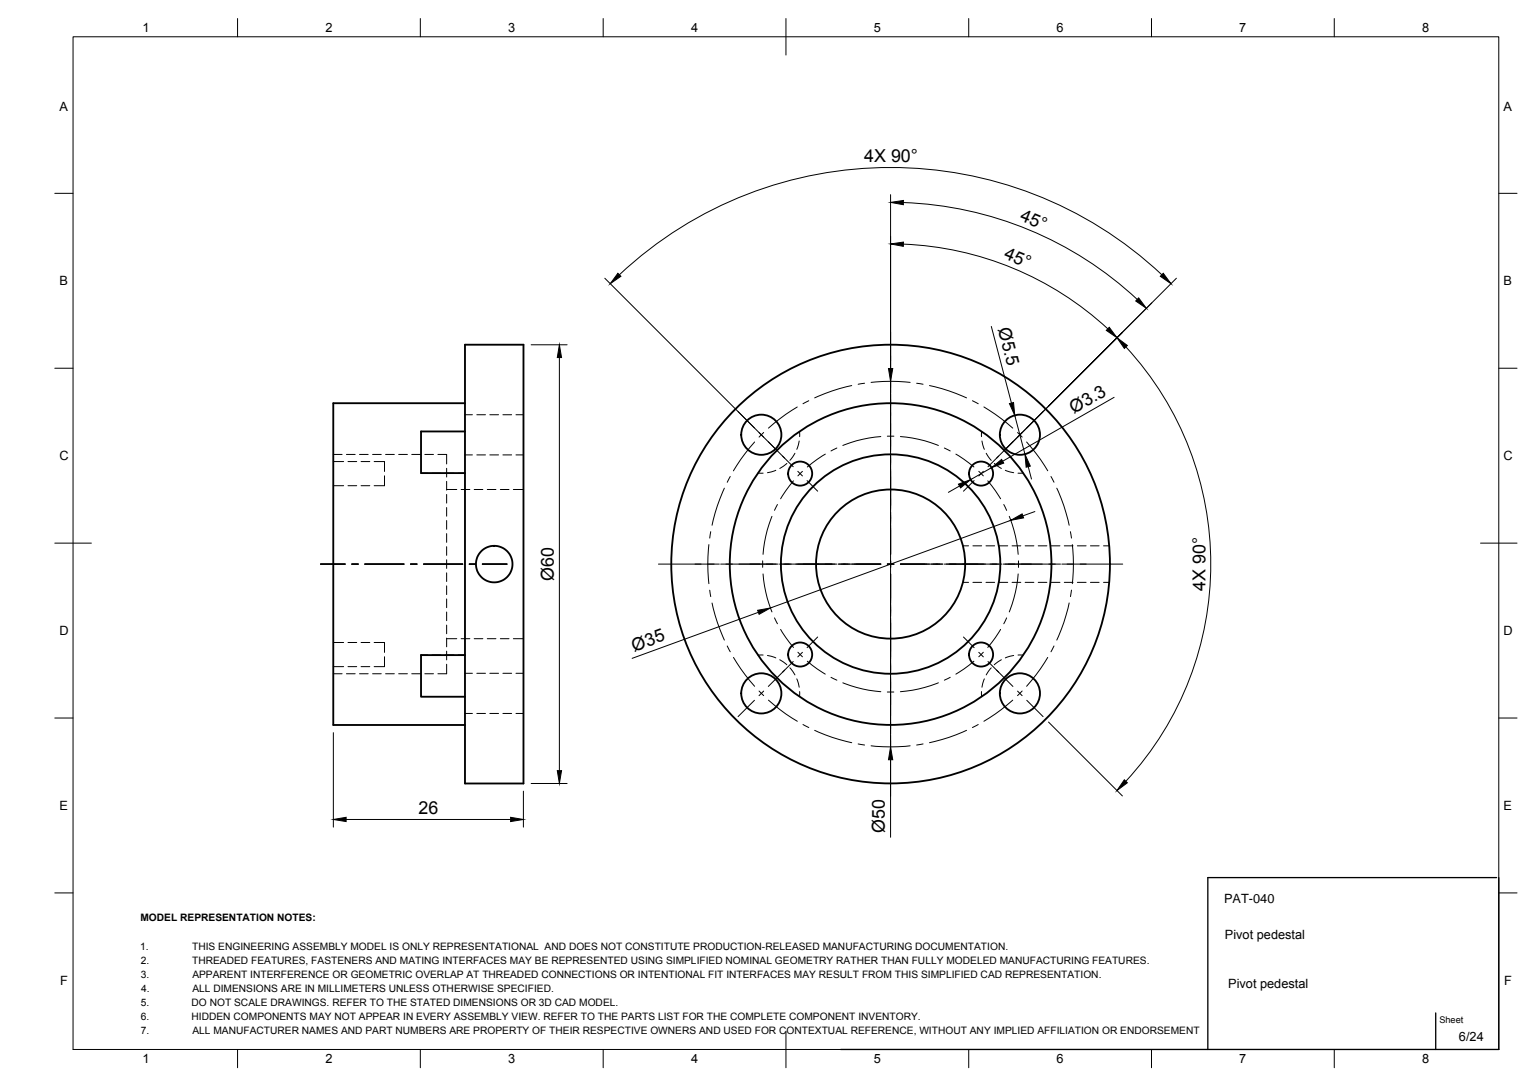
ISO-10303-21;
HEADER;
/* Generated by software containing ST-Developer
 * from STEP Tools, Inc. (www.steptools.com) 
 */

FILE_DESCRIPTION(
/* description */ ('Four-bar tabletop demonstrator'),
/* implementation_level */ '2;1');

FILE_NAME(
/* name */ 'Pivot pedestal.step',
/* time_stamp */ '2026-10-29T17:05:23-07:00',
/* author */ (''),
/* organization */ (''),
/* preprocessor_version */ 'ST-DEVELOPER v20.2',
/* originating_system */ 'Autodesk Translation Framework v15.17.0.0',
/* authorisation */ '');

FILE_SCHEMA (('AUTOMOTIVE_DESIGN { 1 0 10303 214 3 1 1 }'));
ENDSEC;

DATA;
#10=MECHANICAL_DESIGN_GEOMETRIC_PRESENTATION_REPRESENTATION('',(#338),#6705);
#280=B_SPLINE_CURVE_WITH_KNOTS('',3,(#5305,#5306,#5307,#5308,#5309,#5310,
#5311,#5312,#5313,#5314),.UNSPECIFIED.,.F.,.F.,(4,2,2,2,4),(0.,0.0945941824764479,
0.189188364952896,0.283770357603024,0.378352350253152),.UNSPECIFIED.);
#281=B_SPLINE_CURVE_WITH_KNOTS('',3,(#5315,#5316,#5317,#5318,#5319,#5320,
#5321,#5322,#5323,#5324,#5325,#5326,#5327,#5328,#5329,#5330,#5331,#5332,
#5333,#5334,#5335,#5336,#5337,#5338,#5339,#5340),.UNSPECIFIED.,.F.,.F.,
(4,2,2,2,2,2,2,2,2,2,2,2,4),(0.378352350253152,0.47293434290328,0.567516335553408,
0.662110518029855,0.756704700506303,0.851298882982751,0.945893065459199,
1.04047505810933,1.13505705075946,1.22963904340958,1.32422103605971,1.41881521853616,
1.51340940101261),.UNSPECIFIED.);
#282=B_SPLINE_CURVE_WITH_KNOTS('',3,(#5344,#5345,#5346,#5347,#5348,#5349,
#5350,#5351,#5352,#5353,#5354,#5355,#5356,#5357,#5358,#5359,#5360,#5361,
#5362,#5363,#5364,#5365,#5366,#5367,#5368,#5369),.UNSPECIFIED.,.F.,.F.,
(4,2,2,2,2,2,2,2,2,2,2,2,4),(0.,0.0942186410044058,0.188437282008812,0.282655768798837,
0.376874255588861,0.471092742378886,0.565311229168911,0.659529870173317,
0.753748511177723,0.847967152182129,0.942185793186535,1.03640427997656,
1.13062276676658),.UNSPECIFIED.);
#283=B_SPLINE_CURVE_WITH_KNOTS('',3,(#5370,#5371,#5372,#5373,#5374,#5375,
#5376,#5377,#5378,#5379),.UNSPECIFIED.,.F.,.F.,(4,2,2,2,4),(1.13062276676658,
1.22484125355661,1.31905974034663,1.41327838135104,1.50749702235545),
 .UNSPECIFIED.);
#308=SHAPE_REPRESENTATION_RELATIONSHIP('SRR','None',#6814,#323);
#323=ADVANCED_BREP_SHAPE_REPRESENTATION('',(#361),#6687);
#338=STYLED_ITEM('',(#7003),#361);
#361=MANIFOLD_SOLID_BREP('Body1',#3382);
#397=FACE_BOUND('',#814,.T.);
#398=FACE_BOUND('',#815,.T.);
#399=FACE_BOUND('',#816,.T.);
#400=FACE_BOUND('',#817,.T.);
#401=FACE_BOUND('',#818,.T.);
#402=FACE_BOUND('',#825,.T.);
#403=FACE_BOUND('',#827,.T.);
#404=FACE_BOUND('',#829,.T.);
#405=FACE_BOUND('',#831,.T.);
#406=FACE_BOUND('',#832,.T.);
#407=FACE_BOUND('',#833,.T.);
#408=FACE_BOUND('',#834,.T.);
#409=FACE_BOUND('',#835,.T.);
#410=FACE_BOUND('',#837,.T.);
#411=FACE_BOUND('',#838,.T.);
#412=FACE_BOUND('',#839,.T.);
#413=FACE_BOUND('',#840,.T.);
#414=FACE_BOUND('',#841,.T.);
#468=PLANE('',#3610);
#469=PLANE('',#3614);
#470=PLANE('',#3618);
#471=PLANE('',#3622);
#472=PLANE('',#3623);
#473=PLANE('',#3631);
#474=PLANE('',#3636);
#475=PLANE('',#3641);
#476=PLANE('',#3650);
#477=PLANE('',#3667);
#478=PLANE('',#3673);
#479=PLANE('',#3674);
#576=FACE_OUTER_BOUND('',#795,.T.);
#577=FACE_OUTER_BOUND('',#796,.T.);
#578=FACE_OUTER_BOUND('',#797,.T.);
#579=FACE_OUTER_BOUND('',#798,.T.);
#580=FACE_OUTER_BOUND('',#799,.T.);
#581=FACE_OUTER_BOUND('',#800,.T.);
#582=FACE_OUTER_BOUND('',#801,.T.);
#583=FACE_OUTER_BOUND('',#802,.T.);
#584=FACE_OUTER_BOUND('',#803,.T.);
#585=FACE_OUTER_BOUND('',#804,.T.);
#586=FACE_OUTER_BOUND('',#805,.T.);
#587=FACE_OUTER_BOUND('',#806,.T.);
#588=FACE_OUTER_BOUND('',#807,.T.);
#589=FACE_OUTER_BOUND('',#808,.T.);
#590=FACE_OUTER_BOUND('',#809,.T.);
#591=FACE_OUTER_BOUND('',#810,.T.);
#592=FACE_OUTER_BOUND('',#811,.T.);
#593=FACE_OUTER_BOUND('',#812,.T.);
#594=FACE_OUTER_BOUND('',#813,.T.);
#595=FACE_OUTER_BOUND('',#819,.T.);
#596=FACE_OUTER_BOUND('',#820,.T.);
#597=FACE_OUTER_BOUND('',#821,.T.);
#598=FACE_OUTER_BOUND('',#822,.T.);
#599=FACE_OUTER_BOUND('',#823,.T.);
#600=FACE_OUTER_BOUND('',#824,.T.);
#601=FACE_OUTER_BOUND('',#826,.T.);
#602=FACE_OUTER_BOUND('',#828,.T.);
#603=FACE_OUTER_BOUND('',#830,.T.);
#604=FACE_OUTER_BOUND('',#836,.T.);
#795=EDGE_LOOP('',(#2360,#2361,#2362,#2363,#2364,#2365));
#796=EDGE_LOOP('',(#2366,#2367,#2368,#2369));
#797=EDGE_LOOP('',(#2370));
#798=EDGE_LOOP('',(#2371,#2372,#2373,#2374));
#799=EDGE_LOOP('',(#2375));
#800=EDGE_LOOP('',(#2376,#2377,#2378,#2379));
#801=EDGE_LOOP('',(#2380));
#802=EDGE_LOOP('',(#2381,#2382,#2383,#2384));
#803=EDGE_LOOP('',(#2385));
#804=EDGE_LOOP('',(#2386,#2387));
#805=EDGE_LOOP('',(#2388,#2389,#2390,#2391));
#806=EDGE_LOOP('',(#2392,#2393,#2394,#2395));
#807=EDGE_LOOP('',(#2396,#2397));
#808=EDGE_LOOP('',(#2398,#2399,#2400,#2401));
#809=EDGE_LOOP('',(#2402,#2403));
#810=EDGE_LOOP('',(#2404,#2405,#2406,#2407));
#811=EDGE_LOOP('',(#2408,#2409));
#812=EDGE_LOOP('',(#2410,#2411,#2412,#2413,#2414,#2415,#2416,#2417,#2418,
#2419,#2420,#2421,#2422,#2423,#2424,#2425,#2426,#2427,#2428,#2429));
#813=EDGE_LOOP('',(#2430));
#814=EDGE_LOOP('',(#2431,#2432,#2433,#2434,#2435,#2436,#2437,#2438,#2439));
#815=EDGE_LOOP('',(#2440));
#816=EDGE_LOOP('',(#2441));
#817=EDGE_LOOP('',(#2442));
#818=EDGE_LOOP('',(#2443));
#819=EDGE_LOOP('',(#2444,#2445,#2446,#2447));
#820=EDGE_LOOP('',(#2448,#2449,#2450,#2451));
#821=EDGE_LOOP('',(#2452,#2453,#2454,#2455));
#822=EDGE_LOOP('',(#2456,#2457,#2458,#2459));
#823=EDGE_LOOP('',(#2460,#2461,#2462,#2463));
#824=EDGE_LOOP('',(#2464));
#825=EDGE_LOOP('',(#2465));
#826=EDGE_LOOP('',(#2466,#2467,#2468,#2469));
#827=EDGE_LOOP('',(#2470,#2471));
#828=EDGE_LOOP('',(#2472,#2473,#2474,#2475));
#829=EDGE_LOOP('',(#2476,#2477));
#830=EDGE_LOOP('',(#2478));
#831=EDGE_LOOP('',(#2479));
#832=EDGE_LOOP('',(#2480));
#833=EDGE_LOOP('',(#2481));
#834=EDGE_LOOP('',(#2482));
#835=EDGE_LOOP('',(#2483));
#836=EDGE_LOOP('',(#2484));
#837=EDGE_LOOP('',(#2485));
#838=EDGE_LOOP('',(#2486));
#839=EDGE_LOOP('',(#2487));
#840=EDGE_LOOP('',(#2488));
#841=EDGE_LOOP('',(#2489));
#1069=LINE('',#5342,#1239);
#1070=LINE('',#5384,#1240);
#1071=LINE('',#5391,#1241);
#1072=LINE('',#5398,#1242);
#1073=LINE('',#5405,#1243);
#1074=LINE('',#5415,#1244);
#1075=LINE('',#5418,#1245);
#1076=LINE('',#5422,#1246);
#1077=LINE('',#5426,#1247);
#1078=LINE('',#5433,#1248);
#1079=LINE('',#5437,#1249);
#1080=LINE('',#5444,#1250);
#1081=LINE('',#5448,#1251);
#1082=LINE('',#5456,#1252);
#1083=LINE('',#5476,#1253);
#1084=LINE('',#5480,#1254);
#1085=LINE('',#5484,#1255);
#1086=LINE('',#5488,#1256);
#1087=LINE('',#5493,#1257);
#1088=LINE('',#5500,#1258);
#1089=LINE('',#5504,#1259);
#1239=VECTOR('',#4156,0.25);
#1240=VECTOR('',#4161,0.165);
#1241=VECTOR('',#4170,0.165);
#1242=VECTOR('',#4179,0.165);
#1243=VECTOR('',#4188,0.165);
#1244=VECTOR('',#4201,1.);
#1245=VECTOR('',#4204,1.);
#1246=VECTOR('',#4207,1.);
#1247=VECTOR('',#4210,1.);
#1248=VECTOR('',#4219,1.);
#1249=VECTOR('',#4222,1.);
#1250=VECTOR('',#4231,1.);
#1251=VECTOR('',#4234,1.);
#1252=VECTOR('',#4245,2.2);
#1253=VECTOR('',#4272,0.275);
#1254=VECTOR('',#4277,0.275);
#1255=VECTOR('',#4282,0.275);
#1256=VECTOR('',#4287,0.275);
#1257=VECTOR('',#4292,1.5);
#1258=VECTOR('',#4301,3.);
#1259=VECTOR('',#4306,1.02);
#1405=CIRCLE('',#3608,0.165);
#1406=CIRCLE('',#3609,0.165);
#1407=CIRCLE('',#3612,0.165);
#1408=CIRCLE('',#3613,0.165);
#1409=CIRCLE('',#3616,0.165);
#1410=CIRCLE('',#3617,0.165);
#1411=CIRCLE('',#3620,0.165);
#1412=CIRCLE('',#3621,0.165);
#1413=CIRCLE('',#3624,2.2);
#1414=CIRCLE('',#3625,0.525);
#1415=CIRCLE('',#3627,0.525);
#1416=CIRCLE('',#3629,0.525);
#1417=CIRCLE('',#3630,0.525);
#1418=CIRCLE('',#3632,2.2);
#1419=CIRCLE('',#3634,0.525);
#1420=CIRCLE('',#3635,0.525);
#1421=CIRCLE('',#3637,2.2);
#1422=CIRCLE('',#3639,0.525);
#1423=CIRCLE('',#3640,0.525);
#1424=CIRCLE('',#3642,2.2);
#1425=CIRCLE('',#3644,2.2);
#1426=CIRCLE('',#3645,2.2);
#1427=CIRCLE('',#3646,2.2);
#1428=CIRCLE('',#3647,2.2);
#1429=CIRCLE('',#3648,2.2);
#1430=CIRCLE('',#3649,2.2);
#1431=CIRCLE('',#3651,3.);
#1432=CIRCLE('',#3652,0.275);
#1433=CIRCLE('',#3653,0.275);
#1434=CIRCLE('',#3654,0.275);
#1435=CIRCLE('',#3655,0.275);
#1436=CIRCLE('',#3657,0.275);
#1437=CIRCLE('',#3659,0.275);
#1438=CIRCLE('',#3661,0.275);
#1439=CIRCLE('',#3663,0.275);
#1440=CIRCLE('',#3665,1.5);
#1441=CIRCLE('',#3666,1.5);
#1442=CIRCLE('',#3668,1.02);
#1443=CIRCLE('',#3670,3.);
#1444=CIRCLE('',#3672,1.02);
#1624=VERTEX_POINT('',#5303);
#1625=VERTEX_POINT('',#5304);
#1626=VERTEX_POINT('',#5341);
#1627=VERTEX_POINT('',#5343);
#1628=VERTEX_POINT('',#5381);
#1629=VERTEX_POINT('',#5383);
#1630=VERTEX_POINT('',#5388);
#1631=VERTEX_POINT('',#5390);
#1632=VERTEX_POINT('',#5395);
#1633=VERTEX_POINT('',#5397);
#1634=VERTEX_POINT('',#5402);
#1635=VERTEX_POINT('',#5404);
#1636=VERTEX_POINT('',#5409);
#1637=VERTEX_POINT('',#5410);
#1638=VERTEX_POINT('',#5414);
#1639=VERTEX_POINT('',#5416);
#1640=VERTEX_POINT('',#5420);
#1641=VERTEX_POINT('',#5421);
#1642=VERTEX_POINT('',#5423);
#1643=VERTEX_POINT('',#5425);
#1644=VERTEX_POINT('',#5431);
#1645=VERTEX_POINT('',#5432);
#1646=VERTEX_POINT('',#5434);
#1647=VERTEX_POINT('',#5436);
#1648=VERTEX_POINT('',#5442);
#1649=VERTEX_POINT('',#5443);
#1650=VERTEX_POINT('',#5445);
#1651=VERTEX_POINT('',#5447);
#1652=VERTEX_POINT('',#5453);
#1653=VERTEX_POINT('',#5455);
#1654=VERTEX_POINT('',#5463);
#1655=VERTEX_POINT('',#5465);
#1656=VERTEX_POINT('',#5467);
#1657=VERTEX_POINT('',#5469);
#1658=VERTEX_POINT('',#5471);
#1659=VERTEX_POINT('',#5474);
#1660=VERTEX_POINT('',#5478);
#1661=VERTEX_POINT('',#5482);
#1662=VERTEX_POINT('',#5486);
#1663=VERTEX_POINT('',#5490);
#1664=VERTEX_POINT('',#5492);
#1665=VERTEX_POINT('',#5496);
#1666=VERTEX_POINT('',#5499);
#1667=VERTEX_POINT('',#5503);
#1916=EDGE_CURVE('',#1624,#1625,#280,.T.);
#1917=EDGE_CURVE('',#1625,#1624,#281,.T.);
#1918=EDGE_CURVE('',#1625,#1626,#1069,.T.);
#1919=EDGE_CURVE('',#1627,#1626,#282,.T.);
#1920=EDGE_CURVE('',#1626,#1627,#283,.T.);
#1921=EDGE_CURVE('',#1628,#1628,#1405,.T.);
#1922=EDGE_CURVE('',#1628,#1629,#1070,.T.);
#1923=EDGE_CURVE('',#1629,#1629,#1406,.T.);
#1924=EDGE_CURVE('',#1630,#1630,#1407,.T.);
#1925=EDGE_CURVE('',#1630,#1631,#1071,.T.);
#1926=EDGE_CURVE('',#1631,#1631,#1408,.T.);
#1927=EDGE_CURVE('',#1632,#1632,#1409,.T.);
#1928=EDGE_CURVE('',#1632,#1633,#1072,.T.);
#1929=EDGE_CURVE('',#1633,#1633,#1410,.T.);
#1930=EDGE_CURVE('',#1634,#1634,#1411,.T.);
#1931=EDGE_CURVE('',#1634,#1635,#1073,.T.);
#1932=EDGE_CURVE('',#1635,#1635,#1412,.T.);
#1933=EDGE_CURVE('',#1636,#1637,#1413,.T.);
#1934=EDGE_CURVE('',#1637,#1636,#1414,.T.);
#1935=EDGE_CURVE('',#1638,#1636,#1074,.T.);
#1936=EDGE_CURVE('',#1639,#1638,#1415,.T.);
#1937=EDGE_CURVE('',#1637,#1639,#1075,.T.);
#1938=EDGE_CURVE('',#1640,#1641,#1076,.T.);
#1939=EDGE_CURVE('',#1640,#1642,#1416,.T.);
#1940=EDGE_CURVE('',#1643,#1642,#1077,.T.);
#1941=EDGE_CURVE('',#1641,#1643,#1417,.T.);
#1942=EDGE_CURVE('',#1642,#1640,#1418,.T.);
#1943=EDGE_CURVE('',#1644,#1645,#1078,.T.);
#1944=EDGE_CURVE('',#1644,#1646,#1419,.T.);
#1945=EDGE_CURVE('',#1647,#1646,#1079,.T.);
#1946=EDGE_CURVE('',#1645,#1647,#1420,.T.);
#1947=EDGE_CURVE('',#1646,#1644,#1421,.T.);
#1948=EDGE_CURVE('',#1648,#1649,#1080,.T.);
#1949=EDGE_CURVE('',#1648,#1650,#1422,.T.);
#1950=EDGE_CURVE('',#1651,#1650,#1081,.T.);
#1951=EDGE_CURVE('',#1649,#1651,#1423,.T.);
#1952=EDGE_CURVE('',#1650,#1648,#1424,.T.);
#1953=EDGE_CURVE('',#1652,#1652,#1425,.T.);
#1954=EDGE_CURVE('',#1652,#1653,#1082,.T.);
#1955=EDGE_CURVE('',#1653,#1638,#1426,.T.);
#1956=EDGE_CURVE('',#1639,#1651,#1427,.T.);
#1957=EDGE_CURVE('',#1649,#1647,#1428,.T.);
#1958=EDGE_CURVE('',#1645,#1643,#1429,.T.);
#1959=EDGE_CURVE('',#1641,#1653,#1430,.T.);
#1960=EDGE_CURVE('',#1654,#1654,#1431,.T.);
#1961=EDGE_CURVE('',#1655,#1655,#1432,.T.);
#1962=EDGE_CURVE('',#1656,#1656,#1433,.T.);
#1963=EDGE_CURVE('',#1657,#1657,#1434,.T.);
#1964=EDGE_CURVE('',#1658,#1658,#1435,.T.);
#1965=EDGE_CURVE('',#1659,#1659,#1436,.T.);
#1966=EDGE_CURVE('',#1659,#1655,#1083,.T.);
#1967=EDGE_CURVE('',#1660,#1660,#1437,.T.);
#1968=EDGE_CURVE('',#1660,#1658,#1084,.T.);
#1969=EDGE_CURVE('',#1661,#1661,#1438,.T.);
#1970=EDGE_CURVE('',#1661,#1656,#1085,.T.);
#1971=EDGE_CURVE('',#1662,#1662,#1439,.T.);
#1972=EDGE_CURVE('',#1662,#1657,#1086,.T.);
#1973=EDGE_CURVE('',#1663,#1663,#1440,.T.);
#1974=EDGE_CURVE('',#1663,#1664,#1087,.T.);
#1975=EDGE_CURVE('',#1664,#1664,#1441,.T.);
#1976=EDGE_CURVE('',#1665,#1665,#1442,.T.);
#1977=EDGE_CURVE('',#1654,#1666,#1088,.T.);
#1978=EDGE_CURVE('',#1666,#1666,#1443,.T.);
#1979=EDGE_CURVE('',#1665,#1667,#1089,.T.);
#1980=EDGE_CURVE('',#1667,#1667,#1444,.T.);
#2360=ORIENTED_EDGE('',*,*,#1916,.F.);
#2361=ORIENTED_EDGE('',*,*,#1917,.F.);
#2362=ORIENTED_EDGE('',*,*,#1918,.T.);
#2363=ORIENTED_EDGE('',*,*,#1919,.F.);
#2364=ORIENTED_EDGE('',*,*,#1920,.F.);
#2365=ORIENTED_EDGE('',*,*,#1918,.F.);
#2366=ORIENTED_EDGE('',*,*,#1921,.F.);
#2367=ORIENTED_EDGE('',*,*,#1922,.T.);
#2368=ORIENTED_EDGE('',*,*,#1923,.F.);
#2369=ORIENTED_EDGE('',*,*,#1922,.F.);
#2370=ORIENTED_EDGE('',*,*,#1921,.T.);
#2371=ORIENTED_EDGE('',*,*,#1924,.F.);
#2372=ORIENTED_EDGE('',*,*,#1925,.T.);
#2373=ORIENTED_EDGE('',*,*,#1926,.F.);
#2374=ORIENTED_EDGE('',*,*,#1925,.F.);
#2375=ORIENTED_EDGE('',*,*,#1924,.T.);
#2376=ORIENTED_EDGE('',*,*,#1927,.F.);
#2377=ORIENTED_EDGE('',*,*,#1928,.T.);
#2378=ORIENTED_EDGE('',*,*,#1929,.F.);
#2379=ORIENTED_EDGE('',*,*,#1928,.F.);
#2380=ORIENTED_EDGE('',*,*,#1927,.T.);
#2381=ORIENTED_EDGE('',*,*,#1930,.F.);
#2382=ORIENTED_EDGE('',*,*,#1931,.T.);
#2383=ORIENTED_EDGE('',*,*,#1932,.F.);
#2384=ORIENTED_EDGE('',*,*,#1931,.F.);
#2385=ORIENTED_EDGE('',*,*,#1930,.T.);
#2386=ORIENTED_EDGE('',*,*,#1933,.F.);
#2387=ORIENTED_EDGE('',*,*,#1934,.F.);
#2388=ORIENTED_EDGE('',*,*,#1935,.F.);
#2389=ORIENTED_EDGE('',*,*,#1936,.F.);
#2390=ORIENTED_EDGE('',*,*,#1937,.F.);
#2391=ORIENTED_EDGE('',*,*,#1934,.T.);
#2392=ORIENTED_EDGE('',*,*,#1938,.F.);
#2393=ORIENTED_EDGE('',*,*,#1939,.T.);
#2394=ORIENTED_EDGE('',*,*,#1940,.F.);
#2395=ORIENTED_EDGE('',*,*,#1941,.F.);
#2396=ORIENTED_EDGE('',*,*,#1942,.F.);
#2397=ORIENTED_EDGE('',*,*,#1939,.F.);
#2398=ORIENTED_EDGE('',*,*,#1943,.F.);
#2399=ORIENTED_EDGE('',*,*,#1944,.T.);
#2400=ORIENTED_EDGE('',*,*,#1945,.F.);
#2401=ORIENTED_EDGE('',*,*,#1946,.F.);
#2402=ORIENTED_EDGE('',*,*,#1947,.F.);
#2403=ORIENTED_EDGE('',*,*,#1944,.F.);
#2404=ORIENTED_EDGE('',*,*,#1948,.F.);
#2405=ORIENTED_EDGE('',*,*,#1949,.T.);
#2406=ORIENTED_EDGE('',*,*,#1950,.F.);
#2407=ORIENTED_EDGE('',*,*,#1951,.F.);
#2408=ORIENTED_EDGE('',*,*,#1952,.F.);
#2409=ORIENTED_EDGE('',*,*,#1949,.F.);
#2410=ORIENTED_EDGE('',*,*,#1953,.F.);
#2411=ORIENTED_EDGE('',*,*,#1954,.T.);
#2412=ORIENTED_EDGE('',*,*,#1955,.T.);
#2413=ORIENTED_EDGE('',*,*,#1935,.T.);
#2414=ORIENTED_EDGE('',*,*,#1933,.T.);
#2415=ORIENTED_EDGE('',*,*,#1937,.T.);
#2416=ORIENTED_EDGE('',*,*,#1956,.T.);
#2417=ORIENTED_EDGE('',*,*,#1950,.T.);
#2418=ORIENTED_EDGE('',*,*,#1952,.T.);
#2419=ORIENTED_EDGE('',*,*,#1948,.T.);
#2420=ORIENTED_EDGE('',*,*,#1957,.T.);
#2421=ORIENTED_EDGE('',*,*,#1945,.T.);
#2422=ORIENTED_EDGE('',*,*,#1947,.T.);
#2423=ORIENTED_EDGE('',*,*,#1943,.T.);
#2424=ORIENTED_EDGE('',*,*,#1958,.T.);
#2425=ORIENTED_EDGE('',*,*,#1940,.T.);
#2426=ORIENTED_EDGE('',*,*,#1942,.T.);
#2427=ORIENTED_EDGE('',*,*,#1938,.T.);
#2428=ORIENTED_EDGE('',*,*,#1959,.T.);
#2429=ORIENTED_EDGE('',*,*,#1954,.F.);
#2430=ORIENTED_EDGE('',*,*,#1960,.T.);
#2431=ORIENTED_EDGE('',*,*,#1959,.F.);
#2432=ORIENTED_EDGE('',*,*,#1941,.T.);
#2433=ORIENTED_EDGE('',*,*,#1958,.F.);
#2434=ORIENTED_EDGE('',*,*,#1946,.T.);
#2435=ORIENTED_EDGE('',*,*,#1957,.F.);
#2436=ORIENTED_EDGE('',*,*,#1951,.T.);
#2437=ORIENTED_EDGE('',*,*,#1956,.F.);
#2438=ORIENTED_EDGE('',*,*,#1936,.T.);
#2439=ORIENTED_EDGE('',*,*,#1955,.F.);
#2440=ORIENTED_EDGE('',*,*,#1961,.T.);
#2441=ORIENTED_EDGE('',*,*,#1962,.T.);
#2442=ORIENTED_EDGE('',*,*,#1963,.T.);
#2443=ORIENTED_EDGE('',*,*,#1964,.T.);
#2444=ORIENTED_EDGE('',*,*,#1965,.F.);
#2445=ORIENTED_EDGE('',*,*,#1966,.T.);
#2446=ORIENTED_EDGE('',*,*,#1961,.F.);
#2447=ORIENTED_EDGE('',*,*,#1966,.F.);
#2448=ORIENTED_EDGE('',*,*,#1967,.F.);
#2449=ORIENTED_EDGE('',*,*,#1968,.T.);
#2450=ORIENTED_EDGE('',*,*,#1964,.F.);
#2451=ORIENTED_EDGE('',*,*,#1968,.F.);
#2452=ORIENTED_EDGE('',*,*,#1969,.F.);
#2453=ORIENTED_EDGE('',*,*,#1970,.T.);
#2454=ORIENTED_EDGE('',*,*,#1962,.F.);
#2455=ORIENTED_EDGE('',*,*,#1970,.F.);
#2456=ORIENTED_EDGE('',*,*,#1971,.F.);
#2457=ORIENTED_EDGE('',*,*,#1972,.T.);
#2458=ORIENTED_EDGE('',*,*,#1963,.F.);
#2459=ORIENTED_EDGE('',*,*,#1972,.F.);
#2460=ORIENTED_EDGE('',*,*,#1973,.F.);
#2461=ORIENTED_EDGE('',*,*,#1974,.T.);
#2462=ORIENTED_EDGE('',*,*,#1975,.F.);
#2463=ORIENTED_EDGE('',*,*,#1974,.F.);
#2464=ORIENTED_EDGE('',*,*,#1973,.T.);
#2465=ORIENTED_EDGE('',*,*,#1976,.F.);
#2466=ORIENTED_EDGE('',*,*,#1960,.F.);
#2467=ORIENTED_EDGE('',*,*,#1977,.T.);
#2468=ORIENTED_EDGE('',*,*,#1978,.T.);
#2469=ORIENTED_EDGE('',*,*,#1977,.F.);
#2470=ORIENTED_EDGE('',*,*,#1919,.T.);
#2471=ORIENTED_EDGE('',*,*,#1920,.T.);
#2472=ORIENTED_EDGE('',*,*,#1976,.T.);
#2473=ORIENTED_EDGE('',*,*,#1979,.T.);
#2474=ORIENTED_EDGE('',*,*,#1980,.T.);
#2475=ORIENTED_EDGE('',*,*,#1979,.F.);
#2476=ORIENTED_EDGE('',*,*,#1916,.T.);
#2477=ORIENTED_EDGE('',*,*,#1917,.T.);
#2478=ORIENTED_EDGE('',*,*,#1953,.T.);
#2479=ORIENTED_EDGE('',*,*,#1975,.T.);
#2480=ORIENTED_EDGE('',*,*,#1932,.T.);
#2481=ORIENTED_EDGE('',*,*,#1929,.T.);
#2482=ORIENTED_EDGE('',*,*,#1926,.T.);
#2483=ORIENTED_EDGE('',*,*,#1923,.T.);
#2484=ORIENTED_EDGE('',*,*,#1978,.F.);
#2485=ORIENTED_EDGE('',*,*,#1980,.F.);
#2486=ORIENTED_EDGE('',*,*,#1971,.T.);
#2487=ORIENTED_EDGE('',*,*,#1969,.T.);
#2488=ORIENTED_EDGE('',*,*,#1967,.T.);
#2489=ORIENTED_EDGE('',*,*,#1965,.T.);
#3112=CYLINDRICAL_SURFACE('',#3606,0.25);
#3113=CYLINDRICAL_SURFACE('',#3607,0.165);
#3114=CYLINDRICAL_SURFACE('',#3611,0.165);
#3115=CYLINDRICAL_SURFACE('',#3615,0.165);
#3116=CYLINDRICAL_SURFACE('',#3619,0.165);
#3117=CYLINDRICAL_SURFACE('',#3626,0.525);
#3118=CYLINDRICAL_SURFACE('',#3628,0.525);
#3119=CYLINDRICAL_SURFACE('',#3633,0.525);
#3120=CYLINDRICAL_SURFACE('',#3638,0.525);
#3121=CYLINDRICAL_SURFACE('',#3643,2.2);
#3122=CYLINDRICAL_SURFACE('',#3656,0.275);
#3123=CYLINDRICAL_SURFACE('',#3658,0.275);
#3124=CYLINDRICAL_SURFACE('',#3660,0.275);
#3125=CYLINDRICAL_SURFACE('',#3662,0.275);
#3126=CYLINDRICAL_SURFACE('',#3664,1.5);
#3127=CYLINDRICAL_SURFACE('',#3669,3.);
#3128=CYLINDRICAL_SURFACE('',#3671,1.02);
#3192=ADVANCED_FACE('',(#576),#3112,.F.);
#3193=ADVANCED_FACE('',(#577),#3113,.F.);
#3194=ADVANCED_FACE('',(#578),#468,.T.);
#3195=ADVANCED_FACE('',(#579),#3114,.F.);
#3196=ADVANCED_FACE('',(#580),#469,.T.);
#3197=ADVANCED_FACE('',(#581),#3115,.F.);
#3198=ADVANCED_FACE('',(#582),#470,.T.);
#3199=ADVANCED_FACE('',(#583),#3116,.F.);
#3200=ADVANCED_FACE('',(#584),#471,.T.);
#3201=ADVANCED_FACE('',(#585),#472,.F.);
#3202=ADVANCED_FACE('',(#586),#3117,.F.);
#3203=ADVANCED_FACE('',(#587),#3118,.F.);
#3204=ADVANCED_FACE('',(#588),#473,.F.);
#3205=ADVANCED_FACE('',(#589),#3119,.F.);
#3206=ADVANCED_FACE('',(#590),#474,.F.);
#3207=ADVANCED_FACE('',(#591),#3120,.F.);
#3208=ADVANCED_FACE('',(#592),#475,.F.);
#3209=ADVANCED_FACE('',(#593),#3121,.T.);
#3210=ADVANCED_FACE('',(#594,#397,#398,#399,#400,#401),#476,.T.);
#3211=ADVANCED_FACE('',(#595),#3122,.F.);
#3212=ADVANCED_FACE('',(#596),#3123,.F.);
#3213=ADVANCED_FACE('',(#597),#3124,.F.);
#3214=ADVANCED_FACE('',(#598),#3125,.F.);
#3215=ADVANCED_FACE('',(#599),#3126,.F.);
#3216=ADVANCED_FACE('',(#600,#402),#477,.T.);
#3217=ADVANCED_FACE('',(#601,#403),#3127,.T.);
#3218=ADVANCED_FACE('',(#602,#404),#3128,.F.);
#3219=ADVANCED_FACE('',(#603,#405,#406,#407,#408,#409),#478,.T.);
#3220=ADVANCED_FACE('',(#604,#410,#411,#412,#413,#414),#479,.F.);
#3382=CLOSED_SHELL('',(#3192,#3193,#3194,#3195,#3196,#3197,#3198,#3199,
#3200,#3201,#3202,#3203,#3204,#3205,#3206,#3207,#3208,#3209,#3210,#3211,
#3212,#3213,#3214,#3215,#3216,#3217,#3218,#3219,#3220));
#3605=AXIS2_PLACEMENT_3D('',#5301,#4152,#4153);
#3606=AXIS2_PLACEMENT_3D('',#5302,#4154,#4155);
#3607=AXIS2_PLACEMENT_3D('',#5380,#4157,#4158);
#3608=AXIS2_PLACEMENT_3D('',#5382,#4159,#4160);
#3609=AXIS2_PLACEMENT_3D('',#5385,#4162,#4163);
#3610=AXIS2_PLACEMENT_3D('',#5386,#4164,#4165);
#3611=AXIS2_PLACEMENT_3D('',#5387,#4166,#4167);
#3612=AXIS2_PLACEMENT_3D('',#5389,#4168,#4169);
#3613=AXIS2_PLACEMENT_3D('',#5392,#4171,#4172);
#3614=AXIS2_PLACEMENT_3D('',#5393,#4173,#4174);
#3615=AXIS2_PLACEMENT_3D('',#5394,#4175,#4176);
#3616=AXIS2_PLACEMENT_3D('',#5396,#4177,#4178);
#3617=AXIS2_PLACEMENT_3D('',#5399,#4180,#4181);
#3618=AXIS2_PLACEMENT_3D('',#5400,#4182,#4183);
#3619=AXIS2_PLACEMENT_3D('',#5401,#4184,#4185);
#3620=AXIS2_PLACEMENT_3D('',#5403,#4186,#4187);
#3621=AXIS2_PLACEMENT_3D('',#5406,#4189,#4190);
#3622=AXIS2_PLACEMENT_3D('',#5407,#4191,#4192);
#3623=AXIS2_PLACEMENT_3D('',#5408,#4193,#4194);
#3624=AXIS2_PLACEMENT_3D('',#5411,#4195,#4196);
#3625=AXIS2_PLACEMENT_3D('',#5412,#4197,#4198);
#3626=AXIS2_PLACEMENT_3D('',#5413,#4199,#4200);
#3627=AXIS2_PLACEMENT_3D('',#5417,#4202,#4203);
#3628=AXIS2_PLACEMENT_3D('',#5419,#4205,#4206);
#3629=AXIS2_PLACEMENT_3D('',#5424,#4208,#4209);
#3630=AXIS2_PLACEMENT_3D('',#5427,#4211,#4212);
#3631=AXIS2_PLACEMENT_3D('',#5428,#4213,#4214);
#3632=AXIS2_PLACEMENT_3D('',#5429,#4215,#4216);
#3633=AXIS2_PLACEMENT_3D('',#5430,#4217,#4218);
#3634=AXIS2_PLACEMENT_3D('',#5435,#4220,#4221);
#3635=AXIS2_PLACEMENT_3D('',#5438,#4223,#4224);
#3636=AXIS2_PLACEMENT_3D('',#5439,#4225,#4226);
#3637=AXIS2_PLACEMENT_3D('',#5440,#4227,#4228);
#3638=AXIS2_PLACEMENT_3D('',#5441,#4229,#4230);
#3639=AXIS2_PLACEMENT_3D('',#5446,#4232,#4233);
#3640=AXIS2_PLACEMENT_3D('',#5449,#4235,#4236);
#3641=AXIS2_PLACEMENT_3D('',#5450,#4237,#4238);
#3642=AXIS2_PLACEMENT_3D('',#5451,#4239,#4240);
#3643=AXIS2_PLACEMENT_3D('',#5452,#4241,#4242);
#3644=AXIS2_PLACEMENT_3D('',#5454,#4243,#4244);
#3645=AXIS2_PLACEMENT_3D('',#5457,#4246,#4247);
#3646=AXIS2_PLACEMENT_3D('',#5458,#4248,#4249);
#3647=AXIS2_PLACEMENT_3D('',#5459,#4250,#4251);
#3648=AXIS2_PLACEMENT_3D('',#5460,#4252,#4253);
#3649=AXIS2_PLACEMENT_3D('',#5461,#4254,#4255);
#3650=AXIS2_PLACEMENT_3D('',#5462,#4256,#4257);
#3651=AXIS2_PLACEMENT_3D('',#5464,#4258,#4259);
#3652=AXIS2_PLACEMENT_3D('',#5466,#4260,#4261);
#3653=AXIS2_PLACEMENT_3D('',#5468,#4262,#4263);
#3654=AXIS2_PLACEMENT_3D('',#5470,#4264,#4265);
#3655=AXIS2_PLACEMENT_3D('',#5472,#4266,#4267);
#3656=AXIS2_PLACEMENT_3D('',#5473,#4268,#4269);
#3657=AXIS2_PLACEMENT_3D('',#5475,#4270,#4271);
#3658=AXIS2_PLACEMENT_3D('',#5477,#4273,#4274);
#3659=AXIS2_PLACEMENT_3D('',#5479,#4275,#4276);
#3660=AXIS2_PLACEMENT_3D('',#5481,#4278,#4279);
#3661=AXIS2_PLACEMENT_3D('',#5483,#4280,#4281);
#3662=AXIS2_PLACEMENT_3D('',#5485,#4283,#4284);
#3663=AXIS2_PLACEMENT_3D('',#5487,#4285,#4286);
#3664=AXIS2_PLACEMENT_3D('',#5489,#4288,#4289);
#3665=AXIS2_PLACEMENT_3D('',#5491,#4290,#4291);
#3666=AXIS2_PLACEMENT_3D('',#5494,#4293,#4294);
#3667=AXIS2_PLACEMENT_3D('',#5495,#4295,#4296);
#3668=AXIS2_PLACEMENT_3D('',#5497,#4297,#4298);
#3669=AXIS2_PLACEMENT_3D('',#5498,#4299,#4300);
#3670=AXIS2_PLACEMENT_3D('',#5501,#4302,#4303);
#3671=AXIS2_PLACEMENT_3D('',#5502,#4304,#4305);
#3672=AXIS2_PLACEMENT_3D('',#5505,#4307,#4308);
#3673=AXIS2_PLACEMENT_3D('',#5506,#4309,#4310);
#3674=AXIS2_PLACEMENT_3D('',#5507,#4311,#4312);
#4152=DIRECTION('axis',(0.,0.,1.));
#4153=DIRECTION('refdir',(1.,0.,0.));
#4154=DIRECTION('center_axis',(1.,0.,0.));
#4155=DIRECTION('ref_axis',(0.,0.,-1.));
#4156=DIRECTION('',(1.,0.,0.));
#4157=DIRECTION('center_axis',(0.,0.,1.));
#4158=DIRECTION('ref_axis',(1.,0.,0.));
#4159=DIRECTION('center_axis',(0.,0.,1.));
#4160=DIRECTION('ref_axis',(1.,0.,0.));
#4161=DIRECTION('',(0.,0.,1.));
#4162=DIRECTION('center_axis',(0.,0.,-1.));
#4163=DIRECTION('ref_axis',(1.,0.,0.));
#4164=DIRECTION('center_axis',(0.,0.,1.));
#4165=DIRECTION('ref_axis',(1.,0.,0.));
#4166=DIRECTION('center_axis',(0.,0.,1.));
#4167=DIRECTION('ref_axis',(1.,0.,0.));
#4168=DIRECTION('center_axis',(0.,0.,1.));
#4169=DIRECTION('ref_axis',(1.,0.,0.));
#4170=DIRECTION('',(0.,0.,1.));
#4171=DIRECTION('center_axis',(0.,0.,-1.));
#4172=DIRECTION('ref_axis',(1.,0.,0.));
#4173=DIRECTION('center_axis',(0.,0.,1.));
#4174=DIRECTION('ref_axis',(1.,0.,0.));
#4175=DIRECTION('center_axis',(0.,0.,1.));
#4176=DIRECTION('ref_axis',(1.,0.,0.));
#4177=DIRECTION('center_axis',(0.,0.,1.));
#4178=DIRECTION('ref_axis',(1.,0.,0.));
#4179=DIRECTION('',(0.,0.,1.));
#4180=DIRECTION('center_axis',(0.,0.,-1.));
#4181=DIRECTION('ref_axis',(1.,0.,0.));
#4182=DIRECTION('center_axis',(0.,0.,1.));
#4183=DIRECTION('ref_axis',(1.,0.,0.));
#4184=DIRECTION('center_axis',(0.,0.,1.));
#4185=DIRECTION('ref_axis',(1.,0.,0.));
#4186=DIRECTION('center_axis',(0.,0.,1.));
#4187=DIRECTION('ref_axis',(1.,0.,0.));
#4188=DIRECTION('',(0.,0.,1.));
#4189=DIRECTION('center_axis',(0.,0.,-1.));
#4190=DIRECTION('ref_axis',(1.,0.,0.));
#4191=DIRECTION('center_axis',(0.,0.,1.));
#4192=DIRECTION('ref_axis',(1.,0.,0.));
#4193=DIRECTION('center_axis',(0.,0.,1.));
#4194=DIRECTION('ref_axis',(1.,0.,0.));
#4195=DIRECTION('center_axis',(0.,0.,1.));
#4196=DIRECTION('ref_axis',(1.,0.,0.));
#4197=DIRECTION('center_axis',(0.,0.,1.));
#4198=DIRECTION('ref_axis',(1.,0.,0.));
#4199=DIRECTION('center_axis',(0.,0.,1.));
#4200=DIRECTION('ref_axis',(1.,0.,0.));
#4201=DIRECTION('',(0.,0.,1.));
#4202=DIRECTION('center_axis',(0.,0.,1.));
#4203=DIRECTION('ref_axis',(1.,0.,0.));
#4204=DIRECTION('',(0.,0.,-1.));
#4205=DIRECTION('center_axis',(0.,0.,1.));
#4206=DIRECTION('ref_axis',(1.,0.,0.));
#4207=DIRECTION('',(0.,0.,-1.));
#4208=DIRECTION('center_axis',(0.,0.,1.));
#4209=DIRECTION('ref_axis',(1.,0.,0.));
#4210=DIRECTION('',(0.,0.,1.));
#4211=DIRECTION('center_axis',(0.,0.,1.));
#4212=DIRECTION('ref_axis',(1.,0.,0.));
#4213=DIRECTION('center_axis',(0.,0.,1.));
#4214=DIRECTION('ref_axis',(1.,0.,0.));
#4215=DIRECTION('center_axis',(0.,0.,1.));
#4216=DIRECTION('ref_axis',(1.,0.,0.));
#4217=DIRECTION('center_axis',(0.,0.,1.));
#4218=DIRECTION('ref_axis',(-0.707106781186548,-0.707106781186547,0.));
#4219=DIRECTION('',(0.,0.,-1.));
#4220=DIRECTION('center_axis',(0.,0.,1.));
#4221=DIRECTION('ref_axis',(1.,0.,0.));
#4222=DIRECTION('',(0.,0.,1.));
#4223=DIRECTION('center_axis',(0.,0.,1.));
#4224=DIRECTION('ref_axis',(1.,0.,0.));
#4225=DIRECTION('center_axis',(0.,0.,1.));
#4226=DIRECTION('ref_axis',(1.,0.,0.));
#4227=DIRECTION('center_axis',(0.,0.,1.));
#4228=DIRECTION('ref_axis',(1.,0.,0.));
#4229=DIRECTION('center_axis',(0.,0.,1.));
#4230=DIRECTION('ref_axis',(-0.707106781186547,0.707106781186548,0.));
#4231=DIRECTION('',(0.,0.,-1.));
#4232=DIRECTION('center_axis',(0.,0.,1.));
#4233=DIRECTION('ref_axis',(1.,0.,0.));
#4234=DIRECTION('',(0.,0.,1.));
#4235=DIRECTION('center_axis',(0.,0.,1.));
#4236=DIRECTION('ref_axis',(1.,0.,0.));
#4237=DIRECTION('center_axis',(0.,0.,1.));
#4238=DIRECTION('ref_axis',(1.,0.,0.));
#4239=DIRECTION('center_axis',(0.,0.,1.));
#4240=DIRECTION('ref_axis',(1.,0.,0.));
#4241=DIRECTION('center_axis',(0.,0.,1.));
#4242=DIRECTION('ref_axis',(1.,0.,0.));
#4243=DIRECTION('center_axis',(0.,0.,1.));
#4244=DIRECTION('ref_axis',(1.,0.,0.));
#4245=DIRECTION('',(0.,0.,-1.));
#4246=DIRECTION('center_axis',(0.,0.,1.));
#4247=DIRECTION('ref_axis',(1.,0.,0.));
#4248=DIRECTION('center_axis',(0.,0.,1.));
#4249=DIRECTION('ref_axis',(1.,0.,0.));
#4250=DIRECTION('center_axis',(0.,0.,1.));
#4251=DIRECTION('ref_axis',(1.,0.,0.));
#4252=DIRECTION('center_axis',(0.,0.,1.));
#4253=DIRECTION('ref_axis',(1.,0.,0.));
#4254=DIRECTION('center_axis',(0.,0.,1.));
#4255=DIRECTION('ref_axis',(1.,0.,0.));
#4256=DIRECTION('center_axis',(0.,0.,1.));
#4257=DIRECTION('ref_axis',(1.,0.,0.));
#4258=DIRECTION('center_axis',(0.,0.,1.));
#4259=DIRECTION('ref_axis',(1.,0.,0.));
#4260=DIRECTION('center_axis',(0.,0.,-1.));
#4261=DIRECTION('ref_axis',(1.,0.,0.));
#4262=DIRECTION('center_axis',(0.,0.,-1.));
#4263=DIRECTION('ref_axis',(1.,0.,0.));
#4264=DIRECTION('center_axis',(0.,0.,-1.));
#4265=DIRECTION('ref_axis',(1.,0.,0.));
#4266=DIRECTION('center_axis',(0.,0.,-1.));
#4267=DIRECTION('ref_axis',(1.,0.,0.));
#4268=DIRECTION('center_axis',(0.,0.,1.));
#4269=DIRECTION('ref_axis',(1.,0.,0.));
#4270=DIRECTION('center_axis',(0.,0.,1.));
#4271=DIRECTION('ref_axis',(1.,0.,0.));
#4272=DIRECTION('',(0.,0.,1.));
#4273=DIRECTION('center_axis',(0.,0.,1.));
#4274=DIRECTION('ref_axis',(1.,0.,0.));
#4275=DIRECTION('center_axis',(0.,0.,1.));
#4276=DIRECTION('ref_axis',(1.,0.,0.));
#4277=DIRECTION('',(0.,0.,1.));
#4278=DIRECTION('center_axis',(0.,0.,1.));
#4279=DIRECTION('ref_axis',(1.,0.,0.));
#4280=DIRECTION('center_axis',(0.,0.,1.));
#4281=DIRECTION('ref_axis',(1.,0.,0.));
#4282=DIRECTION('',(0.,0.,1.));
#4283=DIRECTION('center_axis',(0.,0.,1.));
#4284=DIRECTION('ref_axis',(1.,0.,0.));
#4285=DIRECTION('center_axis',(0.,0.,1.));
#4286=DIRECTION('ref_axis',(1.,0.,0.));
#4287=DIRECTION('',(0.,0.,1.));
#4288=DIRECTION('center_axis',(0.,0.,1.));
#4289=DIRECTION('ref_axis',(1.,0.,0.));
#4290=DIRECTION('center_axis',(0.,0.,1.));
#4291=DIRECTION('ref_axis',(1.,0.,0.));
#4292=DIRECTION('',(0.,0.,1.));
#4293=DIRECTION('center_axis',(0.,0.,-1.));
#4294=DIRECTION('ref_axis',(1.,0.,0.));
#4295=DIRECTION('center_axis',(0.,0.,1.));
#4296=DIRECTION('ref_axis',(1.,0.,0.));
#4297=DIRECTION('center_axis',(0.,0.,1.));
#4298=DIRECTION('ref_axis',(1.,0.,0.));
#4299=DIRECTION('center_axis',(0.,0.,1.));
#4300=DIRECTION('ref_axis',(1.,0.,0.));
#4301=DIRECTION('',(0.,0.,-1.));
#4302=DIRECTION('center_axis',(0.,0.,1.));
#4303=DIRECTION('ref_axis',(1.,0.,0.));
#4304=DIRECTION('center_axis',(0.,0.,1.));
#4305=DIRECTION('ref_axis',(1.,0.,0.));
#4306=DIRECTION('',(0.,0.,-1.));
#4307=DIRECTION('center_axis',(0.,0.,-1.));
#4308=DIRECTION('ref_axis',(1.,0.,0.));
#4309=DIRECTION('center_axis',(0.,0.,1.));
#4310=DIRECTION('ref_axis',(1.,0.,0.));
#4311=DIRECTION('center_axis',(0.,0.,1.));
#4312=DIRECTION('ref_axis',(1.,0.,0.));
#5301=CARTESIAN_POINT('',(0.,0.,0.));
#5302=CARTESIAN_POINT('Origin',(0.9,0.,1.4));
#5303=CARTESIAN_POINT('',(0.988888264668966,0.25,1.4));
#5304=CARTESIAN_POINT('',(1.02,-1.18386380373883E-17,1.65));
#5305=CARTESIAN_POINT('Ctrl Pts',(0.988888264668966,0.25,1.4));
#5306=CARTESIAN_POINT('Ctrl Pts',(0.988888264668966,0.25,1.43153139415882));
#5307=CARTESIAN_POINT('Ctrl Pts',(0.990553370646674,0.243672048431404,1.46507214966317));
#5308=CARTESIAN_POINT('Ctrl Pts',(0.996491737296663,0.218119830014375,1.52662620974954));
#5309=CARTESIAN_POINT('Ctrl Pts',(1.00067109353237,0.198902128206072,1.5546512623872));
#5310=CARTESIAN_POINT('Ctrl Pts',(1.00845756932386,0.154654113568716,1.59889927702456));
#5311=CARTESIAN_POINT('Ctrl Pts',(1.01258144235289,0.126627870945253,1.61811920309393));
#5312=CARTESIAN_POINT('Ctrl Pts',(1.0183917429657,0.065069600391363,1.64367304400768));
#5313=CARTESIAN_POINT('Ctrl Pts',(1.02,0.031527330883376,1.65));
#5314=CARTESIAN_POINT('Ctrl Pts',(1.02,2.77555756156289E-17,1.65));
#5315=CARTESIAN_POINT('Ctrl Pts',(1.02,6.93889390390723E-18,1.65));
#5316=CARTESIAN_POINT('Ctrl Pts',(1.02,-0.031527330883376,1.65));
#5317=CARTESIAN_POINT('Ctrl Pts',(1.0183917429657,-0.065069600391363,1.64367304400768));
#5318=CARTESIAN_POINT('Ctrl Pts',(1.01258144235289,-0.126627870945253,1.61811920309393));
#5319=CARTESIAN_POINT('Ctrl Pts',(1.00845756932386,-0.154654113568716,1.59889927702456));
#5320=CARTESIAN_POINT('Ctrl Pts',(1.00067109353237,-0.198902128206072,1.5546512623872));
#5321=CARTESIAN_POINT('Ctrl Pts',(0.996491737296663,-0.218119830014375,
1.52662620974954));
#5322=CARTESIAN_POINT('Ctrl Pts',(0.990553370646674,-0.243672048431404,
1.46507214966317));
#5323=CARTESIAN_POINT('Ctrl Pts',(0.988888264668967,-0.25,1.43153139415882));
#5324=CARTESIAN_POINT('Ctrl Pts',(0.988888264668967,-0.25,1.36846860584118));
#5325=CARTESIAN_POINT('Ctrl Pts',(0.990553370646674,-0.243672048431404,
1.33492785033683));
#5326=CARTESIAN_POINT('Ctrl Pts',(0.996491737296663,-0.218119830014375,
1.27337379025046));
#5327=CARTESIAN_POINT('Ctrl Pts',(1.00067109353237,-0.198902128206072,1.2453487376128));
#5328=CARTESIAN_POINT('Ctrl Pts',(1.00845756932386,-0.154654113568716,1.20110072297544));
#5329=CARTESIAN_POINT('Ctrl Pts',(1.01258144235289,-0.126627870945254,1.18188079690607));
#5330=CARTESIAN_POINT('Ctrl Pts',(1.0183917429657,-0.0650696003913633,1.15632695599232));
#5331=CARTESIAN_POINT('Ctrl Pts',(1.02,-0.0315273308833761,1.15));
#5332=CARTESIAN_POINT('Ctrl Pts',(1.02,0.0315273308833759,1.15));
#5333=CARTESIAN_POINT('Ctrl Pts',(1.0183917429657,0.065069600391363,1.15632695599232));
#5334=CARTESIAN_POINT('Ctrl Pts',(1.01258144235289,0.126627870945253,1.18188079690607));
#5335=CARTESIAN_POINT('Ctrl Pts',(1.00845756932386,0.154654113568716,1.20110072297544));
#5336=CARTESIAN_POINT('Ctrl Pts',(1.00067109353237,0.198902128206072,1.2453487376128));
#5337=CARTESIAN_POINT('Ctrl Pts',(0.996491737296663,0.218119830014375,1.27337379025046));
#5338=CARTESIAN_POINT('Ctrl Pts',(0.990553370646674,0.243672048431404,1.33492785033683));
#5339=CARTESIAN_POINT('Ctrl Pts',(0.988888264668967,0.25,1.36846860584118));
#5340=CARTESIAN_POINT('Ctrl Pts',(0.988888264668967,0.25,1.4));
#5341=CARTESIAN_POINT('',(3.,-3.06161699786838E-17,1.65));
#5342=CARTESIAN_POINT('',(0.9,-3.06161699786838E-17,1.65));
#5343=CARTESIAN_POINT('',(2.98956518577535,0.25,1.4));
#5344=CARTESIAN_POINT('Ctrl Pts',(2.98956518577535,0.25,1.4));
#5345=CARTESIAN_POINT('Ctrl Pts',(2.98956518577535,0.25,1.36859378633186));
#5346=CARTESIAN_POINT('Ctrl Pts',(2.99011104995181,0.24372047740942,1.33510417960069));
#5347=CARTESIAN_POINT('Ctrl Pts',(2.99208145165098,0.218202539734559,1.27351367328886));
#5348=CARTESIAN_POINT('Ctrl Pts',(2.99347740802958,0.198964922639276,1.245411532046));
#5349=CARTESIAN_POINT('Ctrl Pts',(2.99609686518216,0.154588504271054,1.20103511367778));
#5350=CARTESIAN_POINT('Ctrl Pts',(2.99749070376198,0.126486346986081,1.18179746841036));
#5351=CARTESIAN_POINT('Ctrl Pts',(2.99945625936844,0.0648957875009219,1.15627950921557));
#5352=CARTESIAN_POINT('Ctrl Pts',(3.,0.0314061622633416,1.15));
#5353=CARTESIAN_POINT('Ctrl Pts',(3.,-0.0314061622633416,1.15));
#5354=CARTESIAN_POINT('Ctrl Pts',(2.99945625936844,-0.0648957875009221,
1.15627950921557));
#5355=CARTESIAN_POINT('Ctrl Pts',(2.99749070376198,-0.126486346986081,1.18179746841036));
#5356=CARTESIAN_POINT('Ctrl Pts',(2.99609686518216,-0.154588504271054,1.20103511367778));
#5357=CARTESIAN_POINT('Ctrl Pts',(2.99347740802958,-0.198964922639276,1.245411532046));
#5358=CARTESIAN_POINT('Ctrl Pts',(2.99208145165098,-0.218202539734559,1.27351367328886));
#5359=CARTESIAN_POINT('Ctrl Pts',(2.99011104995181,-0.24372047740942,1.33510417960069));
#5360=CARTESIAN_POINT('Ctrl Pts',(2.98956518577535,-0.25,1.36859378633186));
#5361=CARTESIAN_POINT('Ctrl Pts',(2.98956518577535,-0.25,1.43140621366814));
#5362=CARTESIAN_POINT('Ctrl Pts',(2.99011104995181,-0.24372047740942,1.4648958203993));
#5363=CARTESIAN_POINT('Ctrl Pts',(2.99208145165098,-0.21820253973456,1.52648632671114));
#5364=CARTESIAN_POINT('Ctrl Pts',(2.99347740802958,-0.198964922639276,1.554588467954));
#5365=CARTESIAN_POINT('Ctrl Pts',(2.99609686518216,-0.154588504271054,1.59896488632222));
#5366=CARTESIAN_POINT('Ctrl Pts',(2.99749070376198,-0.126486346986082,1.61820253158964));
#5367=CARTESIAN_POINT('Ctrl Pts',(2.99945625936844,-0.0648957875009221,
1.64372049078443));
#5368=CARTESIAN_POINT('Ctrl Pts',(3.,-0.0314061622633417,1.65));
#5369=CARTESIAN_POINT('Ctrl Pts',(3.,-5.55111512312578E-17,1.65));
#5370=CARTESIAN_POINT('Ctrl Pts',(3.,-2.08166817117217E-17,1.65));
#5371=CARTESIAN_POINT('Ctrl Pts',(3.,0.0314061622633416,1.65));
#5372=CARTESIAN_POINT('Ctrl Pts',(2.99945625936844,0.0648957875009221,1.64372049078443));
#5373=CARTESIAN_POINT('Ctrl Pts',(2.99749070376198,0.126486346986081,1.61820253158964));
#5374=CARTESIAN_POINT('Ctrl Pts',(2.99609686518216,0.154588504271054,1.59896488632222));
#5375=CARTESIAN_POINT('Ctrl Pts',(2.99347740802958,0.198964922639276,1.554588467954));
#5376=CARTESIAN_POINT('Ctrl Pts',(2.99208145165098,0.218202539734559,1.52648632671114));
#5377=CARTESIAN_POINT('Ctrl Pts',(2.99011104995181,0.24372047740942,1.46489582039931));
#5378=CARTESIAN_POINT('Ctrl Pts',(2.98956518577535,0.25,1.43140621366814));
#5379=CARTESIAN_POINT('Ctrl Pts',(2.98956518577535,0.25,1.4));
#5380=CARTESIAN_POINT('Origin',(-1.23743686707646,-1.23743686707646,2.9));
#5381=CARTESIAN_POINT('',(-1.40243686707646,-1.23743686707646,2.9));
#5382=CARTESIAN_POINT('Origin',(-1.23743686707646,-1.23743686707646,2.9));
#5383=CARTESIAN_POINT('',(-1.40243686707646,-1.23743686707646,3.6));
#5384=CARTESIAN_POINT('',(-1.40243686707646,-1.23743686707646,2.9));
#5385=CARTESIAN_POINT('Origin',(-1.23743686707646,-1.23743686707646,3.6));
#5386=CARTESIAN_POINT('Origin',(-1.23743686707646,-1.23743686707646,2.9));
#5387=CARTESIAN_POINT('Origin',(-1.23743686707646,1.23743686707646,2.9));
#5388=CARTESIAN_POINT('',(-1.40243686707646,1.23743686707646,2.9));
#5389=CARTESIAN_POINT('Origin',(-1.23743686707646,1.23743686707646,2.9));
#5390=CARTESIAN_POINT('',(-1.40243686707646,1.23743686707646,3.6));
#5391=CARTESIAN_POINT('',(-1.40243686707646,1.23743686707646,2.9));
#5392=CARTESIAN_POINT('Origin',(-1.23743686707646,1.23743686707646,3.6));
#5393=CARTESIAN_POINT('Origin',(-1.23743686707646,1.23743686707646,2.9));
#5394=CARTESIAN_POINT('Origin',(1.23743686707646,1.23743686707646,2.9));
#5395=CARTESIAN_POINT('',(1.07243686707646,1.23743686707646,2.9));
#5396=CARTESIAN_POINT('Origin',(1.23743686707646,1.23743686707646,2.9));
#5397=CARTESIAN_POINT('',(1.07243686707646,1.23743686707646,3.6));
#5398=CARTESIAN_POINT('',(1.07243686707646,1.23743686707646,2.9));
#5399=CARTESIAN_POINT('Origin',(1.23743686707646,1.23743686707646,3.6));
#5400=CARTESIAN_POINT('Origin',(1.23743686707646,1.23743686707646,2.9));
#5401=CARTESIAN_POINT('Origin',(1.23743686707646,-1.23743686707646,2.9));
#5402=CARTESIAN_POINT('',(1.07243686707646,-1.23743686707646,2.9));
#5403=CARTESIAN_POINT('Origin',(1.23743686707646,-1.23743686707646,2.9));
#5404=CARTESIAN_POINT('',(1.07243686707646,-1.23743686707646,3.6));
#5405=CARTESIAN_POINT('',(1.07243686707646,-1.23743686707646,2.9));
#5406=CARTESIAN_POINT('Origin',(1.23743686707646,-1.23743686707646,3.6));
#5407=CARTESIAN_POINT('Origin',(1.23743686707646,-1.23743686707646,2.9));
#5408=CARTESIAN_POINT('Origin',(-1.76776695296637,-1.76776695296637,2.4));
#5409=CARTESIAN_POINT('',(-1.8139637388702,-1.24480341984751,2.4));
#5410=CARTESIAN_POINT('',(-1.24480341984751,-1.81396373887019,2.4));
#5411=CARTESIAN_POINT('Origin',(0.,0.,2.4));
#5412=CARTESIAN_POINT('Origin',(-1.76776695296637,-1.76776695296637,2.4));
#5413=CARTESIAN_POINT('Origin',(-1.76776695296637,-1.76776695296637,1.8));
#5414=CARTESIAN_POINT('',(-1.8139637388702,-1.24480341984751,1.8));
#5415=CARTESIAN_POINT('',(-1.8139637388702,-1.24480341984751,1.8));
#5416=CARTESIAN_POINT('',(-1.24480341984751,-1.81396373887019,1.8));
#5417=CARTESIAN_POINT('Origin',(-1.76776695296637,-1.76776695296637,1.8));
#5418=CARTESIAN_POINT('',(-1.24480341984751,-1.81396373887019,1.8));
#5419=CARTESIAN_POINT('Origin',(-1.76776695296637,1.76776695296637,1.8));
#5420=CARTESIAN_POINT('',(-1.81396373887019,1.24480341984751,2.4));
#5421=CARTESIAN_POINT('',(-1.81396373887019,1.24480341984751,1.8));
#5422=CARTESIAN_POINT('',(-1.81396373887019,1.24480341984751,1.8));
#5423=CARTESIAN_POINT('',(-1.24480341984751,1.81396373887019,2.4));
#5424=CARTESIAN_POINT('Origin',(-1.76776695296637,1.76776695296637,2.4));
#5425=CARTESIAN_POINT('',(-1.24480341984751,1.81396373887019,1.8));
#5426=CARTESIAN_POINT('',(-1.24480341984751,1.81396373887019,1.8));
#5427=CARTESIAN_POINT('Origin',(-1.76776695296637,1.76776695296637,1.8));
#5428=CARTESIAN_POINT('Origin',(-1.76776695296637,1.76776695296637,2.4));
#5429=CARTESIAN_POINT('Origin',(0.,0.,2.4));
#5430=CARTESIAN_POINT('Origin',(1.76776695296637,1.76776695296637,1.8));
#5431=CARTESIAN_POINT('',(1.24480341984751,1.81396373887019,2.4));
#5432=CARTESIAN_POINT('',(1.24480341984751,1.81396373887019,1.8));
#5433=CARTESIAN_POINT('',(1.24480341984751,1.81396373887019,1.8));
#5434=CARTESIAN_POINT('',(1.81396373887019,1.24480341984751,2.4));
#5435=CARTESIAN_POINT('Origin',(1.76776695296637,1.76776695296637,2.4));
#5436=CARTESIAN_POINT('',(1.81396373887019,1.24480341984751,1.8));
#5437=CARTESIAN_POINT('',(1.81396373887019,1.24480341984751,1.8));
#5438=CARTESIAN_POINT('Origin',(1.76776695296637,1.76776695296637,1.8));
#5439=CARTESIAN_POINT('Origin',(1.76776695296637,1.76776695296637,2.4));
#5440=CARTESIAN_POINT('Origin',(0.,0.,2.4));
#5441=CARTESIAN_POINT('Origin',(1.76776695296637,-1.76776695296637,1.8));
#5442=CARTESIAN_POINT('',(1.81396373887019,-1.24480341984751,2.4));
#5443=CARTESIAN_POINT('',(1.81396373887019,-1.24480341984751,1.8));
#5444=CARTESIAN_POINT('',(1.81396373887019,-1.24480341984751,1.8));
#5445=CARTESIAN_POINT('',(1.24480341984751,-1.8139637388702,2.4));
#5446=CARTESIAN_POINT('Origin',(1.76776695296637,-1.76776695296637,2.4));
#5447=CARTESIAN_POINT('',(1.24480341984751,-1.8139637388702,1.8));
#5448=CARTESIAN_POINT('',(1.24480341984751,-1.8139637388702,1.8));
#5449=CARTESIAN_POINT('Origin',(1.76776695296637,-1.76776695296637,1.8));
#5450=CARTESIAN_POINT('Origin',(1.76776695296637,-1.76776695296637,2.4));
#5451=CARTESIAN_POINT('Origin',(0.,0.,2.4));
#5452=CARTESIAN_POINT('Origin',(0.,0.,1.));
#5453=CARTESIAN_POINT('',(-2.2,-2.69422295812418E-16,3.6));
#5454=CARTESIAN_POINT('Origin',(0.,0.,3.6));
#5455=CARTESIAN_POINT('',(-2.2,-2.69422295812418E-16,1.8));
#5456=CARTESIAN_POINT('',(-2.2,-2.69422295812418E-16,1.));
#5457=CARTESIAN_POINT('Origin',(0.,0.,1.8));
#5458=CARTESIAN_POINT('Origin',(0.,0.,1.8));
#5459=CARTESIAN_POINT('Origin',(0.,0.,1.8));
#5460=CARTESIAN_POINT('Origin',(0.,0.,1.8));
#5461=CARTESIAN_POINT('Origin',(0.,0.,1.8));
#5462=CARTESIAN_POINT('Origin',(0.,0.,1.8));
#5463=CARTESIAN_POINT('',(-3.,-3.67394039744206E-16,1.8));
#5464=CARTESIAN_POINT('Origin',(0.,0.,1.8));
#5465=CARTESIAN_POINT('',(-2.04276695296637,-1.76776695296637,1.8));
#5466=CARTESIAN_POINT('Origin',(-1.76776695296637,-1.76776695296637,1.8));
#5467=CARTESIAN_POINT('',(1.49276695296637,1.76776695296637,1.8));
#5468=CARTESIAN_POINT('Origin',(1.76776695296637,1.76776695296637,1.8));
#5469=CARTESIAN_POINT('',(1.49276695296637,-1.76776695296637,1.8));
#5470=CARTESIAN_POINT('Origin',(1.76776695296637,-1.76776695296637,1.8));
#5471=CARTESIAN_POINT('',(-2.04276695296637,1.76776695296637,1.8));
#5472=CARTESIAN_POINT('Origin',(-1.76776695296637,1.76776695296637,1.8));
#5473=CARTESIAN_POINT('Origin',(-1.76776695296637,-1.76776695296637,0.9));
#5474=CARTESIAN_POINT('',(-2.04276695296637,-1.76776695296637,1.));
#5475=CARTESIAN_POINT('Origin',(-1.76776695296637,-1.76776695296637,1.));
#5476=CARTESIAN_POINT('',(-2.04276695296637,-1.76776695296637,0.9));
#5477=CARTESIAN_POINT('Origin',(-1.76776695296637,1.76776695296637,0.9));
#5478=CARTESIAN_POINT('',(-2.04276695296637,1.76776695296637,1.));
#5479=CARTESIAN_POINT('Origin',(-1.76776695296637,1.76776695296637,1.));
#5480=CARTESIAN_POINT('',(-2.04276695296637,1.76776695296637,0.9));
#5481=CARTESIAN_POINT('Origin',(1.76776695296637,1.76776695296637,0.9));
#5482=CARTESIAN_POINT('',(1.49276695296637,1.76776695296637,1.));
#5483=CARTESIAN_POINT('Origin',(1.76776695296637,1.76776695296637,1.));
#5484=CARTESIAN_POINT('',(1.49276695296637,1.76776695296637,0.9));
#5485=CARTESIAN_POINT('Origin',(1.76776695296637,-1.76776695296637,0.9));
#5486=CARTESIAN_POINT('',(1.49276695296637,-1.76776695296637,1.));
#5487=CARTESIAN_POINT('Origin',(1.76776695296637,-1.76776695296637,1.));
#5488=CARTESIAN_POINT('',(1.49276695296637,-1.76776695296637,0.9));
#5489=CARTESIAN_POINT('Origin',(0.,0.,2.05));
#5490=CARTESIAN_POINT('',(-1.5,-1.83697019872103E-16,2.05));
#5491=CARTESIAN_POINT('Origin',(0.,0.,2.05));
#5492=CARTESIAN_POINT('',(-1.5,1.83697019872103E-16,3.6));
#5493=CARTESIAN_POINT('',(-1.5,-1.83697019872103E-16,2.05));
#5494=CARTESIAN_POINT('Origin',(0.,0.,3.6));
#5495=CARTESIAN_POINT('Origin',(0.,0.,2.05));
#5496=CARTESIAN_POINT('',(-1.02,-1.2491397351303E-16,2.05));
#5497=CARTESIAN_POINT('Origin',(0.,0.,2.05));
#5498=CARTESIAN_POINT('Origin',(0.,0.,1.));
#5499=CARTESIAN_POINT('',(-3.,-3.67394039744206E-16,1.));
#5500=CARTESIAN_POINT('',(-3.,-3.67394039744206E-16,1.));
#5501=CARTESIAN_POINT('Origin',(0.,0.,1.));
#5502=CARTESIAN_POINT('Origin',(0.,0.,1.));
#5503=CARTESIAN_POINT('',(-1.02,-1.2491397351303E-16,1.));
#5504=CARTESIAN_POINT('',(-1.02,-1.2491397351303E-16,1.));
#5505=CARTESIAN_POINT('Origin',(0.,0.,1.));
#5506=CARTESIAN_POINT('Origin',(0.,0.,3.6));
#5507=CARTESIAN_POINT('Origin',(0.,0.,1.));
#6665=UNCERTAINTY_MEASURE_WITH_UNIT(LENGTH_MEASURE(0.001),#6706,
'DISTANCE_ACCURACY_VALUE',
'Maximum model space distance between geometric entities at asserted c
onnectivities');
#6683=UNCERTAINTY_MEASURE_WITH_UNIT(LENGTH_MEASURE(0.001),#6706,
'DISTANCE_ACCURACY_VALUE',
'Maximum model space distance between geometric entities at asserted c
onnectivities');
#6687=(
GEOMETRIC_REPRESENTATION_CONTEXT(3)
GLOBAL_UNCERTAINTY_ASSIGNED_CONTEXT((#6665))
GLOBAL_UNIT_ASSIGNED_CONTEXT((#6706,#6708,#6709))
REPRESENTATION_CONTEXT('','3D')
);
#6705=(
GEOMETRIC_REPRESENTATION_CONTEXT(3)
GLOBAL_UNCERTAINTY_ASSIGNED_CONTEXT((#6683))
GLOBAL_UNIT_ASSIGNED_CONTEXT((#6706,#6708,#6709))
REPRESENTATION_CONTEXT('','3D')
);
#6706=(
LENGTH_UNIT()
NAMED_UNIT(*)
SI_UNIT(.CENTI.,.METRE.)
);
#6708=(
NAMED_UNIT(*)
PLANE_ANGLE_UNIT()
SI_UNIT($,.RADIAN.)
);
#6709=(
NAMED_UNIT(*)
SI_UNIT($,.STERADIAN.)
SOLID_ANGLE_UNIT()
);
#6713=SHAPE_DEFINITION_REPRESENTATION(#6734,#6814);
#6734=PRODUCT_DEFINITION_SHAPE('',$,#6836);
#6814=SHAPE_REPRESENTATION('',(#3605),#6687);
#6832=PRODUCT_DEFINITION_CONTEXT('part definition',#6897,'design');
#6836=PRODUCT_DEFINITION('Pivot pedestal','Pivot pedestal',#6857,#6832);
#6857=PRODUCT_DEFINITION_FORMATION('',$,#6902);
#6897=APPLICATION_CONTEXT(
'Core Data for Automotive Mechanical Design Process');
#6898=PRODUCT_CONTEXT('part definition',#6897,'mechanical');
#6902=PRODUCT('Pivot pedestal','Pivot pedestal','Pivot pedestal',(#6898));
#6997=COLOUR_RGB('Off White',0.89,0.88,0.83);
#6998=FILL_AREA_STYLE_COLOUR('',#6997);
#6999=FILL_AREA_STYLE('',(#6998));
#7000=SURFACE_STYLE_FILL_AREA(#6999);
#7001=SURFACE_SIDE_STYLE('',(#7000));
#7002=SURFACE_STYLE_USAGE(.BOTH.,#7001);
#7003=PRESENTATION_STYLE_ASSIGNMENT((#7002));
ENDSEC;
END-ISO-10303-21;
